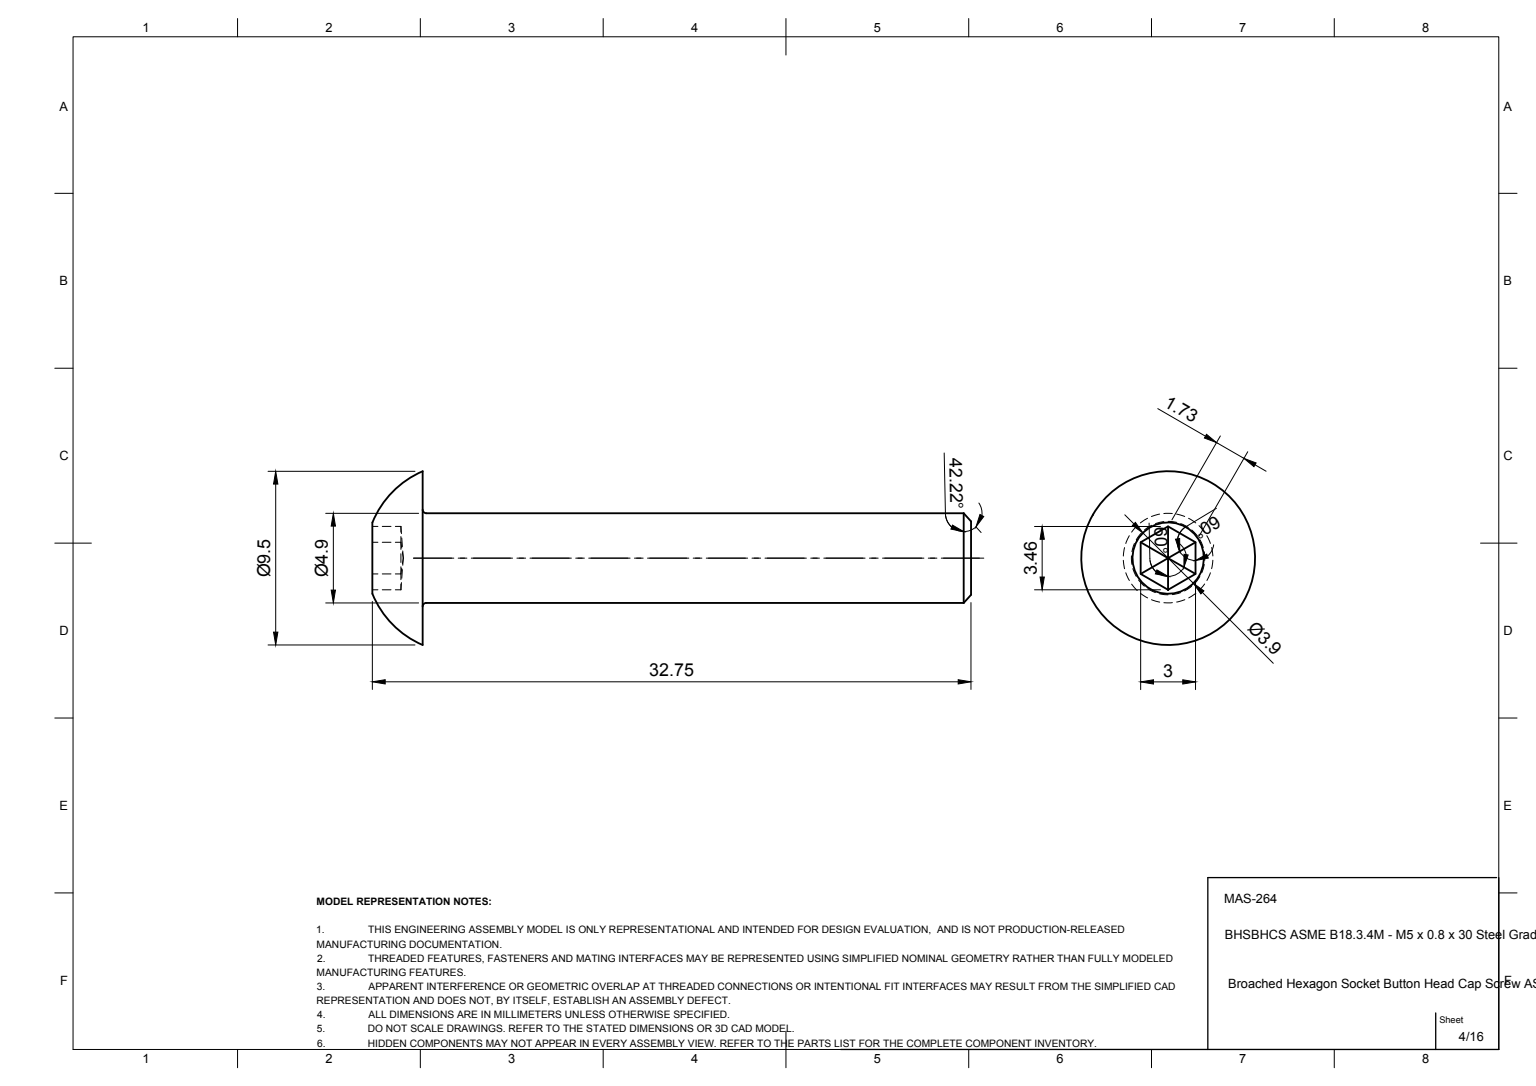
ISO-10303-21;
HEADER;
/* Generated by software containing ST-Developer
 * from STEP Tools, Inc. (www.steptools.com) 
 */

FILE_DESCRIPTION(
/* description */ (''),
/* implementation_level */ '2;1');

FILE_NAME(
/* name */ 'BHSBHCS ASME B18.3.4M - M5 x 0.8 x 30 Steel Grade 2 Plain.step',
/* time_stamp */ '2026-10-12T15:37:13-07:00',
/* author */ (''),
/* organization */ (''),
/* preprocessor_version */ 'ST-DEVELOPER v20.2',
/* originating_system */ 'Autodesk Translation Framework v15.15.0.0',
/* authorisation */ '');

FILE_SCHEMA (('AUTOMOTIVE_DESIGN { 1 0 10303 214 3 1 1 }'));
ENDSEC;

DATA;
#10=MECHANICAL_DESIGN_GEOMETRIC_PRESENTATION_REPRESENTATION('',(#357),#36460);
#105=SPHERICAL_SURFACE('',#12419,5.16792277674902);
#118=SHAPE_REPRESENTATION_RELATIONSHIP('SRR','None',#36530,#131);
#131=ADVANCED_BREP_SHAPE_REPRESENTATION('',(#389),#36459);
#263=FACE_BOUND('',#2370,.T.);
#264=FACE_BOUND('',#2386,.T.);
#325=CONICAL_SURFACE('',#12394,2.27961999999998,0.833832411830472);
#357=STYLED_ITEM('',(#36596),#389);
#389=MANIFOLD_SOLID_BREP('Body1',#11293);
#699=PLANE('',#12401);
#700=PLANE('',#12404);
#701=PLANE('',#12405);
#702=PLANE('',#12406);
#703=PLANE('',#12407);
#704=PLANE('',#12408);
#705=PLANE('',#12409);
#706=PLANE('',#12410);
#707=PLANE('',#12411);
#708=PLANE('',#12412);
#709=PLANE('',#12413);
#710=PLANE('',#12414);
#711=PLANE('',#12415);
#712=PLANE('',#12416);
#713=PLANE('',#12417);
#1026=TOROIDAL_SURFACE('',#12397,2.6505,0.2);
#1622=FACE_OUTER_BOUND('',#2367,.T.);
#1623=FACE_OUTER_BOUND('',#2368,.T.);
#1624=FACE_OUTER_BOUND('',#2369,.T.);
#1625=FACE_OUTER_BOUND('',#2371,.T.);
#1626=FACE_OUTER_BOUND('',#2372,.T.);
#1627=FACE_OUTER_BOUND('',#2373,.T.);
#1628=FACE_OUTER_BOUND('',#2374,.T.);
#1629=FACE_OUTER_BOUND('',#2375,.T.);
#1630=FACE_OUTER_BOUND('',#2376,.T.);
#1631=FACE_OUTER_BOUND('',#2377,.T.);
#1632=FACE_OUTER_BOUND('',#2378,.T.);
#1633=FACE_OUTER_BOUND('',#2379,.T.);
#1634=FACE_OUTER_BOUND('',#2380,.T.);
#1635=FACE_OUTER_BOUND('',#2381,.T.);
#1636=FACE_OUTER_BOUND('',#2382,.T.);
#1637=FACE_OUTER_BOUND('',#2383,.T.);
#1638=FACE_OUTER_BOUND('',#2384,.T.);
#1639=FACE_OUTER_BOUND('',#2385,.T.);
#1640=FACE_OUTER_BOUND('',#2387,.T.);
#2367=EDGE_LOOP('',(#10346,#10347,#10348,#10349));
#2368=EDGE_LOOP('',(#10350,#10351,#10352,#10353));
#2369=EDGE_LOOP('',(#10354));
#2370=EDGE_LOOP('',(#10355));
#2371=EDGE_LOOP('',(#10356,#10357,#10358,#10359));
#2372=EDGE_LOOP('',(#10360,#10361,#10362));
#2373=EDGE_LOOP('',(#10363,#10364,#10365));
#2374=EDGE_LOOP('',(#10366,#10367,#10368));
#2375=EDGE_LOOP('',(#10369,#10370,#10371));
#2376=EDGE_LOOP('',(#10372,#10373,#10374));
#2377=EDGE_LOOP('',(#10375,#10376,#10377));
#2378=EDGE_LOOP('',(#10378,#10379,#10380,#10381));
#2379=EDGE_LOOP('',(#10382,#10383,#10384,#10385));
#2380=EDGE_LOOP('',(#10386,#10387,#10388,#10389));
#2381=EDGE_LOOP('',(#10390,#10391,#10392,#10393));
#2382=EDGE_LOOP('',(#10394,#10395,#10396,#10397));
#2383=EDGE_LOOP('',(#10398,#10399,#10400,#10401));
#2384=EDGE_LOOP('',(#10402));
#2385=EDGE_LOOP('',(#10403));
#2386=EDGE_LOOP('',(#10404,#10405,#10406,#10407,#10408,#10409));
#2387=EDGE_LOOP('',(#10410,#10411,#10412,#10413));
#3308=LINE('',#36345,#4254);
#3309=LINE('',#36357,#4255);
#3310=LINE('',#36361,#4256);
#3311=LINE('',#36363,#4257);
#3312=LINE('',#36364,#4258);
#3313=LINE('',#36367,#4259);
#3314=LINE('',#36368,#4260);
#3315=LINE('',#36371,#4261);
#3316=LINE('',#36372,#4262);
#3317=LINE('',#36375,#4263);
#3318=LINE('',#36376,#4264);
#3319=LINE('',#36379,#4265);
#3320=LINE('',#36380,#4266);
#3321=LINE('',#36382,#4267);
#3322=LINE('',#36386,#4268);
#3323=LINE('',#36387,#4269);
#3324=LINE('',#36388,#4270);
#3325=LINE('',#36391,#4271);
#3326=LINE('',#36392,#4272);
#3327=LINE('',#36395,#4273);
#3328=LINE('',#36396,#4274);
#3329=LINE('',#36399,#4275);
#3330=LINE('',#36400,#4276);
#3331=LINE('',#36403,#4277);
#3332=LINE('',#36404,#4278);
#3333=LINE('',#36406,#4279);
#4254=VECTOR('',#15273,2.27961999999998);
#4255=VECTOR('',#15290,2.4505);
#4256=VECTOR('',#15293,9.99999999999999);
#4257=VECTOR('',#15294,10.);
#4258=VECTOR('',#15295,10.);
#4259=VECTOR('',#15298,10.);
#4260=VECTOR('',#15299,10.);
#4261=VECTOR('',#15302,10.);
#4262=VECTOR('',#15303,9.99999999999999);
#4263=VECTOR('',#15306,10.);
#4264=VECTOR('',#15307,10.);
#4265=VECTOR('',#15310,10.);
#4266=VECTOR('',#15311,10.);
#4267=VECTOR('',#15314,10.);
#4268=VECTOR('',#15317,10.);
#4269=VECTOR('',#15318,10.);
#4270=VECTOR('',#15319,10.);
#4271=VECTOR('',#15322,10.);
#4272=VECTOR('',#15323,10.);
#4273=VECTOR('',#15326,10.);
#4274=VECTOR('',#15327,10.);
#4275=VECTOR('',#15330,10.);
#4276=VECTOR('',#15331,10.);
#4277=VECTOR('',#15334,10.);
#4278=VECTOR('',#15335,10.);
#4279=VECTOR('',#15338,10.);
#4585=CIRCLE('',#12395,2.4505);
#4586=CIRCLE('',#12396,2.00924000000001);
#4587=CIRCLE('',#12398,2.4505);
#4588=CIRCLE('',#12399,0.2);
#4589=CIRCLE('',#12400,2.6505);
#4590=CIRCLE('',#12402,4.75);
#4591=CIRCLE('',#12418,1.95);
#4592=CIRCLE('',#12420,5.16792277674902);
#5631=VERTEX_POINT('',#36342);
#5632=VERTEX_POINT('',#36344);
#5633=VERTEX_POINT('',#36348);
#5634=VERTEX_POINT('',#36350);
#5635=VERTEX_POINT('',#36354);
#5636=VERTEX_POINT('',#36359);
#5637=VERTEX_POINT('',#36360);
#5638=VERTEX_POINT('',#36362);
#5639=VERTEX_POINT('',#36366);
#5640=VERTEX_POINT('',#36370);
#5641=VERTEX_POINT('',#36374);
#5642=VERTEX_POINT('',#36378);
#5643=VERTEX_POINT('',#36384);
#5644=VERTEX_POINT('',#36385);
#5645=VERTEX_POINT('',#36390);
#5646=VERTEX_POINT('',#36394);
#5647=VERTEX_POINT('',#36398);
#5648=VERTEX_POINT('',#36402);
#5649=VERTEX_POINT('',#36409);
#7204=EDGE_CURVE('',#5631,#5631,#4585,.T.);
#7205=EDGE_CURVE('',#5631,#5632,#3308,.T.);
#7206=EDGE_CURVE('',#5632,#5632,#4586,.T.);
#7207=EDGE_CURVE('',#5633,#5633,#4587,.T.);
#7208=EDGE_CURVE('',#5633,#5634,#4588,.T.);
#7209=EDGE_CURVE('',#5634,#5634,#4589,.T.);
#7210=EDGE_CURVE('',#5635,#5635,#4590,.T.);
#7211=EDGE_CURVE('',#5631,#5633,#3309,.T.);
#7212=EDGE_CURVE('',#5636,#5637,#3310,.T.);
#7213=EDGE_CURVE('',#5638,#5636,#3311,.T.);
#7214=EDGE_CURVE('',#5638,#5637,#3312,.T.);
#7215=EDGE_CURVE('',#5639,#5638,#3313,.T.);
#7216=EDGE_CURVE('',#5639,#5637,#3314,.T.);
#7217=EDGE_CURVE('',#5640,#5639,#3315,.T.);
#7218=EDGE_CURVE('',#5640,#5637,#3316,.T.);
#7219=EDGE_CURVE('',#5641,#5640,#3317,.T.);
#7220=EDGE_CURVE('',#5641,#5637,#3318,.T.);
#7221=EDGE_CURVE('',#5642,#5641,#3319,.T.);
#7222=EDGE_CURVE('',#5642,#5637,#3320,.T.);
#7223=EDGE_CURVE('',#5636,#5642,#3321,.T.);
#7224=EDGE_CURVE('',#5643,#5644,#3322,.T.);
#7225=EDGE_CURVE('',#5643,#5638,#3323,.T.);
#7226=EDGE_CURVE('',#5644,#5636,#3324,.T.);
#7227=EDGE_CURVE('',#5645,#5643,#3325,.T.);
#7228=EDGE_CURVE('',#5645,#5639,#3326,.T.);
#7229=EDGE_CURVE('',#5646,#5645,#3327,.T.);
#7230=EDGE_CURVE('',#5646,#5640,#3328,.T.);
#7231=EDGE_CURVE('',#5647,#5646,#3329,.T.);
#7232=EDGE_CURVE('',#5647,#5641,#3330,.T.);
#7233=EDGE_CURVE('',#5648,#5647,#3331,.T.);
#7234=EDGE_CURVE('',#5648,#5642,#3332,.T.);
#7235=EDGE_CURVE('',#5644,#5648,#3333,.T.);
#7236=EDGE_CURVE('',#5649,#5649,#4591,.T.);
#7237=EDGE_CURVE('',#5649,#5635,#4592,.T.);
#10346=ORIENTED_EDGE('',*,*,#7204,.F.);
#10347=ORIENTED_EDGE('',*,*,#7205,.T.);
#10348=ORIENTED_EDGE('',*,*,#7206,.F.);
#10349=ORIENTED_EDGE('',*,*,#7205,.F.);
#10350=ORIENTED_EDGE('',*,*,#7207,.T.);
#10351=ORIENTED_EDGE('',*,*,#7208,.T.);
#10352=ORIENTED_EDGE('',*,*,#7209,.T.);
#10353=ORIENTED_EDGE('',*,*,#7208,.F.);
#10354=ORIENTED_EDGE('',*,*,#7210,.T.);
#10355=ORIENTED_EDGE('',*,*,#7209,.F.);
#10356=ORIENTED_EDGE('',*,*,#7204,.T.);
#10357=ORIENTED_EDGE('',*,*,#7211,.T.);
#10358=ORIENTED_EDGE('',*,*,#7207,.F.);
#10359=ORIENTED_EDGE('',*,*,#7211,.F.);
#10360=ORIENTED_EDGE('',*,*,#7212,.F.);
#10361=ORIENTED_EDGE('',*,*,#7213,.F.);
#10362=ORIENTED_EDGE('',*,*,#7214,.T.);
#10363=ORIENTED_EDGE('',*,*,#7214,.F.);
#10364=ORIENTED_EDGE('',*,*,#7215,.F.);
#10365=ORIENTED_EDGE('',*,*,#7216,.T.);
#10366=ORIENTED_EDGE('',*,*,#7216,.F.);
#10367=ORIENTED_EDGE('',*,*,#7217,.F.);
#10368=ORIENTED_EDGE('',*,*,#7218,.T.);
#10369=ORIENTED_EDGE('',*,*,#7218,.F.);
#10370=ORIENTED_EDGE('',*,*,#7219,.F.);
#10371=ORIENTED_EDGE('',*,*,#7220,.T.);
#10372=ORIENTED_EDGE('',*,*,#7220,.F.);
#10373=ORIENTED_EDGE('',*,*,#7221,.F.);
#10374=ORIENTED_EDGE('',*,*,#7222,.T.);
#10375=ORIENTED_EDGE('',*,*,#7222,.F.);
#10376=ORIENTED_EDGE('',*,*,#7223,.F.);
#10377=ORIENTED_EDGE('',*,*,#7212,.T.);
#10378=ORIENTED_EDGE('',*,*,#7224,.F.);
#10379=ORIENTED_EDGE('',*,*,#7225,.T.);
#10380=ORIENTED_EDGE('',*,*,#7213,.T.);
#10381=ORIENTED_EDGE('',*,*,#7226,.F.);
#10382=ORIENTED_EDGE('',*,*,#7227,.F.);
#10383=ORIENTED_EDGE('',*,*,#7228,.T.);
#10384=ORIENTED_EDGE('',*,*,#7215,.T.);
#10385=ORIENTED_EDGE('',*,*,#7225,.F.);
#10386=ORIENTED_EDGE('',*,*,#7229,.F.);
#10387=ORIENTED_EDGE('',*,*,#7230,.T.);
#10388=ORIENTED_EDGE('',*,*,#7217,.T.);
#10389=ORIENTED_EDGE('',*,*,#7228,.F.);
#10390=ORIENTED_EDGE('',*,*,#7231,.F.);
#10391=ORIENTED_EDGE('',*,*,#7232,.T.);
#10392=ORIENTED_EDGE('',*,*,#7219,.T.);
#10393=ORIENTED_EDGE('',*,*,#7230,.F.);
#10394=ORIENTED_EDGE('',*,*,#7233,.F.);
#10395=ORIENTED_EDGE('',*,*,#7234,.T.);
#10396=ORIENTED_EDGE('',*,*,#7221,.T.);
#10397=ORIENTED_EDGE('',*,*,#7232,.F.);
#10398=ORIENTED_EDGE('',*,*,#7235,.F.);
#10399=ORIENTED_EDGE('',*,*,#7226,.T.);
#10400=ORIENTED_EDGE('',*,*,#7223,.T.);
#10401=ORIENTED_EDGE('',*,*,#7234,.F.);
#10402=ORIENTED_EDGE('',*,*,#7206,.T.);
#10403=ORIENTED_EDGE('',*,*,#7236,.F.);
#10404=ORIENTED_EDGE('',*,*,#7224,.T.);
#10405=ORIENTED_EDGE('',*,*,#7235,.T.);
#10406=ORIENTED_EDGE('',*,*,#7233,.T.);
#10407=ORIENTED_EDGE('',*,*,#7231,.T.);
#10408=ORIENTED_EDGE('',*,*,#7229,.T.);
#10409=ORIENTED_EDGE('',*,*,#7227,.T.);
#10410=ORIENTED_EDGE('',*,*,#7236,.T.);
#10411=ORIENTED_EDGE('',*,*,#7237,.T.);
#10412=ORIENTED_EDGE('',*,*,#7210,.F.);
#10413=ORIENTED_EDGE('',*,*,#7237,.F.);
#10647=CYLINDRICAL_SURFACE('',#12403,2.4505);
#11243=ADVANCED_FACE('',(#1622),#325,.T.);
#11244=ADVANCED_FACE('',(#1623),#1026,.F.);
#11245=ADVANCED_FACE('',(#1624,#263),#699,.T.);
#11246=ADVANCED_FACE('',(#1625),#10647,.T.);
#11247=ADVANCED_FACE('',(#1626),#700,.F.);
#11248=ADVANCED_FACE('',(#1627),#701,.F.);
#11249=ADVANCED_FACE('',(#1628),#702,.F.);
#11250=ADVANCED_FACE('',(#1629),#703,.F.);
#11251=ADVANCED_FACE('',(#1630),#704,.F.);
#11252=ADVANCED_FACE('',(#1631),#705,.F.);
#11253=ADVANCED_FACE('',(#1632),#706,.F.);
#11254=ADVANCED_FACE('',(#1633),#707,.F.);
#11255=ADVANCED_FACE('',(#1634),#708,.F.);
#11256=ADVANCED_FACE('',(#1635),#709,.F.);
#11257=ADVANCED_FACE('',(#1636),#710,.F.);
#11258=ADVANCED_FACE('',(#1637),#711,.F.);
#11259=ADVANCED_FACE('',(#1638),#712,.T.);
#11260=ADVANCED_FACE('',(#1639,#264),#713,.T.);
#11261=ADVANCED_FACE('',(#1640),#105,.T.);
#11293=CLOSED_SHELL('',(#11243,#11244,#11245,#11246,#11247,#11248,#11249,
#11250,#11251,#11252,#11253,#11254,#11255,#11256,#11257,#11258,#11259,#11260,
#11261));
#12393=AXIS2_PLACEMENT_3D('',#36340,#15267,#15268);
#12394=AXIS2_PLACEMENT_3D('',#36341,#15269,#15270);
#12395=AXIS2_PLACEMENT_3D('',#36343,#15271,#15272);
#12396=AXIS2_PLACEMENT_3D('',#36346,#15274,#15275);
#12397=AXIS2_PLACEMENT_3D('',#36347,#15276,#15277);
#12398=AXIS2_PLACEMENT_3D('',#36349,#15278,#15279);
#12399=AXIS2_PLACEMENT_3D('',#36351,#15280,#15281);
#12400=AXIS2_PLACEMENT_3D('',#36352,#15282,#15283);
#12401=AXIS2_PLACEMENT_3D('',#36353,#15284,#15285);
#12402=AXIS2_PLACEMENT_3D('',#36355,#15286,#15287);
#12403=AXIS2_PLACEMENT_3D('',#36356,#15288,#15289);
#12404=AXIS2_PLACEMENT_3D('',#36358,#15291,#15292);
#12405=AXIS2_PLACEMENT_3D('',#36365,#15296,#15297);
#12406=AXIS2_PLACEMENT_3D('',#36369,#15300,#15301);
#12407=AXIS2_PLACEMENT_3D('',#36373,#15304,#15305);
#12408=AXIS2_PLACEMENT_3D('',#36377,#15308,#15309);
#12409=AXIS2_PLACEMENT_3D('',#36381,#15312,#15313);
#12410=AXIS2_PLACEMENT_3D('',#36383,#15315,#15316);
#12411=AXIS2_PLACEMENT_3D('',#36389,#15320,#15321);
#12412=AXIS2_PLACEMENT_3D('',#36393,#15324,#15325);
#12413=AXIS2_PLACEMENT_3D('',#36397,#15328,#15329);
#12414=AXIS2_PLACEMENT_3D('',#36401,#15332,#15333);
#12415=AXIS2_PLACEMENT_3D('',#36405,#15336,#15337);
#12416=AXIS2_PLACEMENT_3D('',#36407,#15339,#15340);
#12417=AXIS2_PLACEMENT_3D('',#36408,#15341,#15342);
#12418=AXIS2_PLACEMENT_3D('',#36410,#15343,#15344);
#12419=AXIS2_PLACEMENT_3D('',#36411,#15345,#15346);
#12420=AXIS2_PLACEMENT_3D('',#36412,#15347,#15348);
#15267=DIRECTION('axis',(0.,0.,1.));
#15268=DIRECTION('refdir',(1.,0.,0.));
#15269=DIRECTION('center_axis',(2.75333173930341E-16,0.,1.));
#15270=DIRECTION('ref_axis',(-1.,0.,2.75333173930341E-16));
#15271=DIRECTION('center_axis',(2.75333173930341E-16,0.,1.));
#15272=DIRECTION('ref_axis',(-1.,0.,2.75333173930341E-16));
#15273=DIRECTION('',(-0.740512347492959,-9.06866076086345E-17,-0.672042754004882));
#15274=DIRECTION('center_axis',(-2.75333173930341E-16,0.,-1.));
#15275=DIRECTION('ref_axis',(-1.,0.,2.75333173930341E-16));
#15276=DIRECTION('center_axis',(-2.75333173930341E-16,0.,-1.));
#15277=DIRECTION('ref_axis',(-1.,0.,2.72638525605195E-16));
#15278=DIRECTION('center_axis',(2.75333173930341E-16,0.,1.));
#15279=DIRECTION('ref_axis',(-1.,0.,2.75333173930341E-16));
#15280=DIRECTION('center_axis',(1.22464679914735E-16,1.,-3.37185890152874E-32));
#15281=DIRECTION('ref_axis',(1.,-1.22464679914735E-16,-2.79941343255335E-16));
#15282=DIRECTION('center_axis',(-2.75333173930341E-16,0.,-1.));
#15283=DIRECTION('ref_axis',(-1.,0.,2.75333173930341E-16));
#15284=DIRECTION('center_axis',(-2.75333173930341E-16,0.,-1.));
#15285=DIRECTION('ref_axis',(-1.,0.,2.75333173930341E-16));
#15286=DIRECTION('center_axis',(-2.75333173930341E-16,0.,-1.));
#15287=DIRECTION('ref_axis',(1.,0.,-2.75333173930341E-16));
#15288=DIRECTION('center_axis',(-2.75333173930341E-16,0.,-1.));
#15289=DIRECTION('ref_axis',(-1.,0.,2.75333173930341E-16));
#15290=DIRECTION('',(2.75333173930341E-16,0.,1.));
#15291=DIRECTION('center_axis',(0.0435778713738291,-0.0754790873051733,
-0.996194698091746));
#15292=DIRECTION('ref_axis',(-0.866025403784439,-0.5,-3.35810244624808E-17));
#15293=DIRECTION('',(0.,0.997141949694316,-0.0755508581011305));
#15294=DIRECTION('',(-0.866025403784439,-0.5,0.));
#15295=DIRECTION('',(-0.863550259614423,0.498570974847158,-0.0755508581011305));
#15296=DIRECTION('center_axis',(0.0871557427476581,0.,-0.996194698091746));
#15297=DIRECTION('ref_axis',(0.,-1.,0.));
#15298=DIRECTION('',(0.,-1.,0.));
#15299=DIRECTION('',(-0.863550259614423,-0.498570974847158,-0.0755508581011305));
#15300=DIRECTION('center_axis',(0.0435778713738291,0.0754790873051733,-0.996194698091746));
#15301=DIRECTION('ref_axis',(0.866025403784439,-0.5,3.35810244624808E-17));
#15302=DIRECTION('',(0.866025403784439,-0.5,0.));
#15303=DIRECTION('',(-1.59381164582915E-16,-0.997141949694316,-0.0755508581011305));
#15304=DIRECTION('center_axis',(-0.0435778713738291,0.0754790873051733,
-0.996194698091746));
#15305=DIRECTION('ref_axis',(0.866025403784439,0.5,-3.35810244624808E-17));
#15306=DIRECTION('',(0.866025403784439,0.5,0.));
#15307=DIRECTION('',(0.863550259614423,-0.498570974847159,-0.0755508581011305));
#15308=DIRECTION('center_axis',(-0.0871557427476581,5.58657470692638E-17,
-0.996194698091746));
#15309=DIRECTION('ref_axis',(6.40987562127855E-16,1.,-3.92662944814522E-32));
#15310=DIRECTION('',(6.40987562127855E-16,1.,0.));
#15311=DIRECTION('',(0.863550259614423,0.498570974847158,-0.0755508581011305));
#15312=DIRECTION('center_axis',(-0.0435778713738291,-0.0754790873051733,
-0.996194698091746));
#15313=DIRECTION('ref_axis',(-0.866025403784439,0.5,3.35810244624808E-17));
#15314=DIRECTION('',(-0.866025403784439,0.5,0.));
#15315=DIRECTION('center_axis',(0.5,-0.866025403784439,0.));
#15316=DIRECTION('ref_axis',(-0.866025403784439,-0.5,0.));
#15317=DIRECTION('',(-0.866025403784439,-0.5,2.38445523128275E-16));
#15318=DIRECTION('',(0.,0.,-1.));
#15319=DIRECTION('',(0.,0.,-1.));
#15320=DIRECTION('center_axis',(1.,0.,0.));
#15321=DIRECTION('ref_axis',(0.,-1.,0.));
#15322=DIRECTION('',(0.,-1.,0.));
#15323=DIRECTION('',(0.,0.,-1.));
#15324=DIRECTION('center_axis',(0.5,0.866025403784439,0.));
#15325=DIRECTION('ref_axis',(0.866025403784439,-0.5,0.));
#15326=DIRECTION('',(0.866025403784439,-0.5,-2.38445523128275E-16));
#15327=DIRECTION('',(0.,0.,-1.));
#15328=DIRECTION('center_axis',(-0.5,0.866025403784439,0.));
#15329=DIRECTION('ref_axis',(0.866025403784439,0.5,0.));
#15330=DIRECTION('',(0.866025403784439,0.5,-2.38445523128275E-16));
#15331=DIRECTION('',(0.,0.,-1.));
#15332=DIRECTION('center_axis',(-1.,6.40987562127855E-16,0.));
#15333=DIRECTION('ref_axis',(6.40987562127855E-16,1.,0.));
#15334=DIRECTION('',(6.40987562127855E-16,1.,-1.76485139930534E-31));
#15335=DIRECTION('',(0.,0.,-1.));
#15336=DIRECTION('center_axis',(-0.5,-0.866025403784439,0.));
#15337=DIRECTION('ref_axis',(-0.866025403784439,0.5,0.));
#15338=DIRECTION('',(-0.866025403784439,0.5,2.38445523128275E-16));
#15339=DIRECTION('center_axis',(-2.75333173930341E-16,0.,-1.));
#15340=DIRECTION('ref_axis',(-1.,0.,2.75333173930341E-16));
#15341=DIRECTION('center_axis',(2.75333173930341E-16,0.,1.));
#15342=DIRECTION('ref_axis',(1.,0.,-2.75333173930341E-16));
#15343=DIRECTION('center_axis',(-2.75333173930341E-16,0.,-1.));
#15344=DIRECTION('ref_axis',(1.,0.,-2.75333173930341E-16));
#15345=DIRECTION('center_axis',(1.22464679914735E-16,0.,1.));
#15346=DIRECTION('ref_axis',(1.,0.,-8.59318587050222E-17));
#15347=DIRECTION('center_axis',(1.22464679914735E-16,-1.,-7.49879891330929E-33));
#15348=DIRECTION('ref_axis',(-1.,-1.22464679914735E-16,5.37074116906389E-17));
#36340=CARTESIAN_POINT('',(0.,0.,0.));
#36341=CARTESIAN_POINT('Origin',(-8.06355459534025E-15,0.,-29.75462));
#36342=CARTESIAN_POINT('',(2.45049999999999,3.00099698131059E-16,-29.599539985206));
#36343=CARTESIAN_POINT('Origin',(-8.02085592265385E-15,0.,-29.599539985206));
#36344=CARTESIAN_POINT('',(2.00924,-2.46060933471884E-16,-30.));
#36345=CARTESIAN_POINT('',(2.27961999999997,2.79172933627226E-16,-29.75462));
#36346=CARTESIAN_POINT('Origin',(-8.13111584955928E-15,0.,-30.));
#36347=CARTESIAN_POINT('Origin',(7.38127335647334E-17,0.,-0.200000000000542));
#36348=CARTESIAN_POINT('',(2.4505,3.00099698131059E-16,-0.200000000000543));
#36349=CARTESIAN_POINT('Origin',(7.38127335647334E-17,0.,-0.200000000000542));
#36350=CARTESIAN_POINT('',(2.6505,-3.24592634114006E-16,-5.43004329167852E-13));
#36351=CARTESIAN_POINT('Origin',(2.6505,-3.24592634114006E-16,-0.200000000000543));
#36352=CARTESIAN_POINT('Origin',(1.28879368350801E-16,0.,-5.4227455859035E-13));
#36353=CARTESIAN_POINT('Origin',(-2.5,0.,-5.41596033937917E-13));
#36354=CARTESIAN_POINT('',(-4.75,0.,-1.02889918807136E-12));
#36355=CARTESIAN_POINT('Origin',(1.28879368350667E-16,0.,-1.03020702064753E-12));
#36356=CARTESIAN_POINT('Origin',(-4.00111824060424E-15,0.,-15.0000000000003));
#36357=CARTESIAN_POINT('',(2.4505,-3.00099698131059E-16,-15.0000000000003));
#36358=CARTESIAN_POINT('Origin',(2.77555756156289E-16,-1.73205080756888,
1.19));
#36359=CARTESIAN_POINT('',(2.77555756156289E-16,-1.73205080756888,1.19));
#36360=CARTESIAN_POINT('',(4.16333634234434E-16,-1.11022302462516E-15,1.05876700471111));
#36361=CARTESIAN_POINT('',(4.16333634234434E-16,-1.3015097128034,1.15737901843634));
#36362=CARTESIAN_POINT('',(1.5,-0.866025403784439,1.19));
#36363=CARTESIAN_POINT('',(2.67440770322657E-16,-1.73205080756888,1.19));
#36364=CARTESIAN_POINT('',(1.12714047455993,-0.650754856401699,1.15737901843634));
#36365=CARTESIAN_POINT('Origin',(1.5,-0.866025403784439,1.19));
#36366=CARTESIAN_POINT('',(1.5,0.866025403784438,1.19));
#36367=CARTESIAN_POINT('',(1.5,-0.866025403784439,1.19));
#36368=CARTESIAN_POINT('',(1.12714047455993,0.650754856401699,1.15737901843634));
#36369=CARTESIAN_POINT('Origin',(1.5,0.866025403784438,1.19));
#36370=CARTESIAN_POINT('',(0.,1.73205080756888,1.19));
#36371=CARTESIAN_POINT('',(1.5,0.866025403784438,1.19));
#36372=CARTESIAN_POINT('',(-2.77555756156289E-16,1.3015097128034,1.15737901843634));
#36373=CARTESIAN_POINT('Origin',(0.,1.73205080756888,1.19));
#36374=CARTESIAN_POINT('',(-1.5,0.866025403784439,1.19));
#36375=CARTESIAN_POINT('',(-6.93889390390723E-17,1.73205080756888,1.19));
#36376=CARTESIAN_POINT('',(-1.12714047455993,0.6507548564017,1.15737901843634));
#36377=CARTESIAN_POINT('Origin',(-1.5,0.866025403784439,1.19));
#36378=CARTESIAN_POINT('',(-1.5,-0.866025403784438,1.19));
#36379=CARTESIAN_POINT('',(-1.5,0.866025403784439,1.19));
#36380=CARTESIAN_POINT('',(-1.12714047455993,-0.650754856401698,1.15737901843634));
#36381=CARTESIAN_POINT('Origin',(-1.5,-0.866025403784438,1.19));
#36382=CARTESIAN_POINT('',(-1.5,-0.866025403784438,1.19));
#36383=CARTESIAN_POINT('Origin',(1.5,-0.866025403784439,2.75));
#36384=CARTESIAN_POINT('',(1.5,-0.866025403784439,2.75));
#36385=CARTESIAN_POINT('',(2.77555756156289E-16,-1.73205080756888,2.75));
#36386=CARTESIAN_POINT('',(0.393750000000001,-1.50471913907546,2.74999999999968));
#36387=CARTESIAN_POINT('',(1.5,-0.866025403784439,2.75));
#36388=CARTESIAN_POINT('',(2.77555756156289E-16,-1.73205080756888,2.75));
#36389=CARTESIAN_POINT('Origin',(1.5,0.866025403784438,2.75));
#36390=CARTESIAN_POINT('',(1.5,0.866025403784438,2.75));
#36391=CARTESIAN_POINT('',(1.5,0.433012701892219,2.74999999999967));
#36392=CARTESIAN_POINT('',(1.5,0.866025403784438,2.75));
#36393=CARTESIAN_POINT('Origin',(0.,1.73205080756888,2.75));
#36394=CARTESIAN_POINT('',(-6.93889390390723E-17,1.73205080756888,2.75));
#36395=CARTESIAN_POINT('',(-0.35625,1.93773184096768,2.74999999999968));
#36396=CARTESIAN_POINT('',(-6.93889390390723E-17,1.73205080756888,2.75));
#36397=CARTESIAN_POINT('Origin',(-1.5,0.866025403784439,2.75));
#36398=CARTESIAN_POINT('',(-1.5,0.866025403784439,2.75));
#36399=CARTESIAN_POINT('',(-1.85625,0.660344370385635,2.74999999999968));
#36400=CARTESIAN_POINT('',(-1.5,0.866025403784439,2.75));
#36401=CARTESIAN_POINT('Origin',(-1.5,-0.866025403784438,2.75));
#36402=CARTESIAN_POINT('',(-1.5,-0.866025403784438,2.75));
#36403=CARTESIAN_POINT('',(-1.5,-0.433012701892219,2.74999999999968));
#36404=CARTESIAN_POINT('',(-1.5,-0.866025403784438,2.75));
#36405=CARTESIAN_POINT('Origin',(2.77555756156289E-16,-1.73205080756888,
2.75));
#36406=CARTESIAN_POINT('',(-1.10625,-1.09335707227785,2.74999999999968));
#36407=CARTESIAN_POINT('Origin',(-8.04911692853238E-15,0.,-30.));
#36408=CARTESIAN_POINT('Origin',(-1.95,0.,2.74999999999968));
#36409=CARTESIAN_POINT('',(-1.95,0.,2.74999999999968));
#36410=CARTESIAN_POINT('Origin',(8.86045596659299E-16,0.,2.74999999999968));
#36411=CARTESIAN_POINT('Origin',(-5.55111512312578E-16,0.,-2.03590909090889));
#36412=CARTESIAN_POINT('Origin',(-5.55111512312578E-16,0.,-2.03590909090889));
#36443=UNCERTAINTY_MEASURE_WITH_UNIT(LENGTH_MEASURE(0.01),#36461,
'DISTANCE_ACCURACY_VALUE',
'Maximum model space distance between geometric entities at asserted c
onnectivities');
#36444=UNCERTAINTY_MEASURE_WITH_UNIT(LENGTH_MEASURE(0.01),#36461,
'DISTANCE_ACCURACY_VALUE',
'Maximum model space distance between geometric entities at asserted c
onnectivities');
#36459=(
GEOMETRIC_REPRESENTATION_CONTEXT(3)
GLOBAL_UNCERTAINTY_ASSIGNED_CONTEXT((#36443))
GLOBAL_UNIT_ASSIGNED_CONTEXT((#36461,#36463,#36464))
REPRESENTATION_CONTEXT('','3D')
);
#36460=(
GEOMETRIC_REPRESENTATION_CONTEXT(3)
GLOBAL_UNCERTAINTY_ASSIGNED_CONTEXT((#36444))
GLOBAL_UNIT_ASSIGNED_CONTEXT((#36461,#36463,#36464))
REPRESENTATION_CONTEXT('','3D')
);
#36461=(
LENGTH_UNIT()
NAMED_UNIT(*)
SI_UNIT(.MILLI.,.METRE.)
);
#36463=(
NAMED_UNIT(*)
PLANE_ANGLE_UNIT()
SI_UNIT($,.RADIAN.)
);
#36464=(
NAMED_UNIT(*)
SI_UNIT($,.STERADIAN.)
SOLID_ANGLE_UNIT()
);
#36479=SHAPE_DEFINITION_REPRESENTATION(#36499,#36530);
#36499=PRODUCT_DEFINITION_SHAPE('',$,#36546);
#36530=SHAPE_REPRESENTATION('',(#12393),#36459);
#36531=PRODUCT_DEFINITION_CONTEXT('part definition',#36578,'design');
#36546=PRODUCT_DEFINITION(
'BHSBHCS ASME B18.3.4M - M5 x 0.8 x 30 Steel Grade 2 Plain',
'BHSBHCS ASME B18.3.4M - M5 x 0.8 x 30 Steel Grade 2 Plain',#36561,#36531);
#36561=PRODUCT_DEFINITION_FORMATION('',$,#36594);
#36578=APPLICATION_CONTEXT(
'Core Data for Automotive Mechanical Design Process');
#36579=PRODUCT_CONTEXT('part definition',#36578,'mechanical');
#36594=PRODUCT(
'BHSBHCS ASME B18.3.4M - M5 x 0.8 x 30 Steel Grade 2 Plain',
'BHSBHCS ASME B18.3.4M - M5 x 0.8 x 30 Steel Grade 2 Plain',
'Broached Hexagon Socket Button Head Cap Screw ASME B18.3.4M - M5 x 0.
8 x 30',(#36579));
#36596=PRESENTATION_STYLE_ASSIGNMENT((#36601));
#36601=SURFACE_STYLE_USAGE(.BOTH.,#36606);
#36606=SURFACE_SIDE_STYLE('',(#36611));
#36611=SURFACE_STYLE_FILL_AREA(#36616);
#36616=FILL_AREA_STYLE('Opaque(160,160,160)',(#36621));
#36621=FILL_AREA_STYLE_COLOUR('Opaque(160,160,160)',#36626);
#36626=COLOUR_RGB('Opaque(160,160,160)', 0.09019608, 0.27058824, 0.51372549);
ENDSEC;
END-ISO-10303-21;
